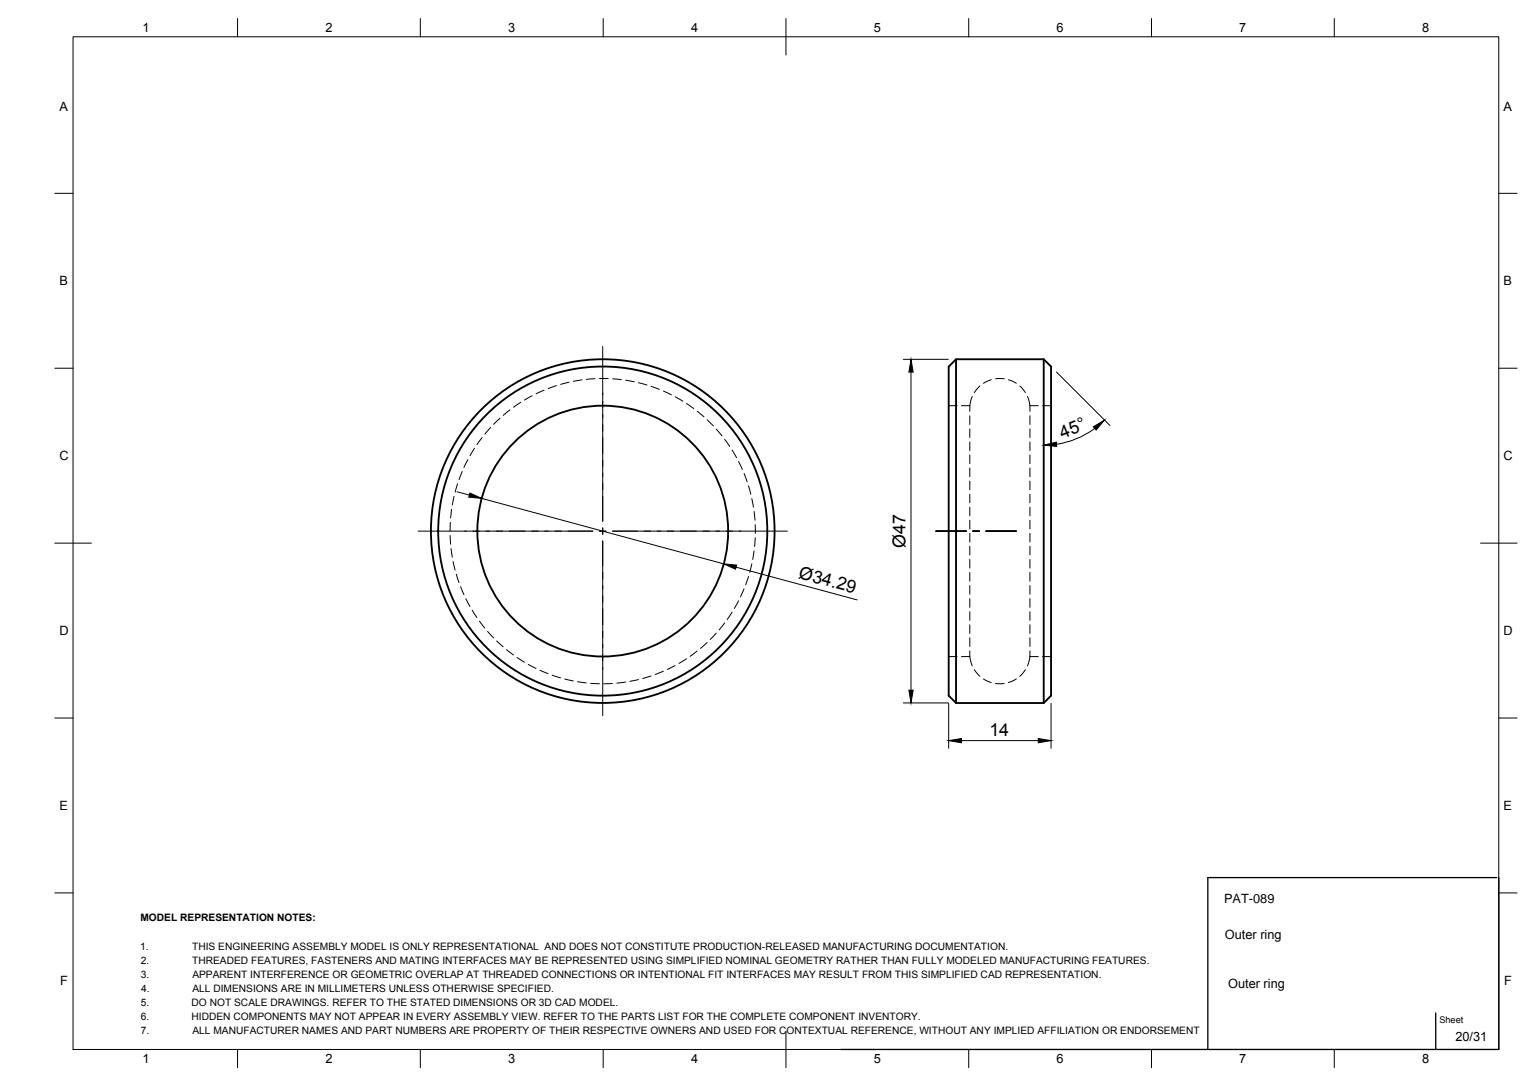
ISO-10303-21;
HEADER;
/* Generated by software containing ST-Developer
 * from STEP Tools, Inc. (www.steptools.com) 
 */

FILE_DESCRIPTION(
/* description */ ('Rotary union on bearing shaft'),
/* implementation_level */ '2;1');

FILE_NAME(
/* name */ 'Outer ring.step',
/* time_stamp */ '2026-10-28T03:24:01-07:00',
/* author */ (''),
/* organization */ (''),
/* preprocessor_version */ 'ST-DEVELOPER v20.2',
/* originating_system */ 'Autodesk Translation Framework v15.17.0.0',
/* authorisation */ '');

FILE_SCHEMA (('AUTOMOTIVE_DESIGN { 1 0 10303 214 3 1 1 }'));
ENDSEC;

DATA;
#10=MECHANICAL_DESIGN_GEOMETRIC_PRESENTATION_REPRESENTATION('',(#325),#9448);
#203=CONICAL_SURFACE('',#5460,2.3,0.785398163397449);
#204=CONICAL_SURFACE('',#5464,2.3,0.785398163397449);
#224=TOROIDAL_SURFACE('',#5449,1.675,0.412776);
#271=SHAPE_REPRESENTATION_RELATIONSHIP('SRR','None',#9572,#298);
#298=ADVANCED_BREP_SHAPE_REPRESENTATION('',(#360),#9432);
#325=STYLED_ITEM('',(#9778),#360);
#360=MANIFOLD_SOLID_BREP('Body1',#4880);
#446=FACE_BOUND('',#1143,.T.);
#447=FACE_BOUND('',#1148,.T.);
#552=PLANE('',#5457);
#553=PLANE('',#5466);
#775=FACE_OUTER_BOUND('',#1140,.T.);
#776=FACE_OUTER_BOUND('',#1141,.T.);
#777=FACE_OUTER_BOUND('',#1142,.T.);
#778=FACE_OUTER_BOUND('',#1144,.T.);
#779=FACE_OUTER_BOUND('',#1145,.T.);
#780=FACE_OUTER_BOUND('',#1146,.T.);
#781=FACE_OUTER_BOUND('',#1147,.T.);
#782=FACE_OUTER_BOUND('',#1149,.T.);
#1140=EDGE_LOOP('',(#3755,#3756,#3757,#3758,#3759,#3760));
#1141=EDGE_LOOP('',(#3761,#3762,#3763,#3764,#3765));
#1142=EDGE_LOOP('',(#3766));
#1143=EDGE_LOOP('',(#3767));
#1144=EDGE_LOOP('',(#3768,#3769,#3770,#3771));
#1145=EDGE_LOOP('',(#3772,#3773,#3774,#3775));
#1146=EDGE_LOOP('',(#3776,#3777,#3778,#3779));
#1147=EDGE_LOOP('',(#3780));
#1148=EDGE_LOOP('',(#3781));
#1149=EDGE_LOOP('',(#3782,#3783,#3784,#3785,#3786));
#1487=LINE('',#8078,#1807);
#1488=LINE('',#8087,#1808);
#1489=LINE('',#8091,#1809);
#1490=LINE('',#8095,#1810);
#1491=LINE('',#8098,#1811);
#1807=VECTOR('',#6460,1.71469);
#1808=VECTOR('',#6471,2.3);
#1809=VECTOR('',#6476,2.35);
#1810=VECTOR('',#6481,2.3);
#1811=VECTOR('',#6486,1.71469);
#2111=CIRCLE('',#5450,1.71469);
#2112=CIRCLE('',#5451,1.71469);
#2113=CIRCLE('',#5452,0.412776);
#2114=CIRCLE('',#5453,1.71469);
#2115=CIRCLE('',#5454,1.71469);
#2116=CIRCLE('',#5456,1.71469);
#2117=CIRCLE('',#5458,2.25);
#2118=CIRCLE('',#5459,1.71469);
#2119=CIRCLE('',#5461,2.35);
#2120=CIRCLE('',#5463,2.35);
#2121=CIRCLE('',#5465,2.25);
#2414=VERTEX_POINT('',#8066);
#2415=VERTEX_POINT('',#8067);
#2416=VERTEX_POINT('',#8070);
#2417=VERTEX_POINT('',#8072);
#2418=VERTEX_POINT('',#8076);
#2419=VERTEX_POINT('',#8080);
#2420=VERTEX_POINT('',#8082);
#2421=VERTEX_POINT('',#8085);
#2422=VERTEX_POINT('',#8089);
#2423=VERTEX_POINT('',#8093);
#2905=EDGE_CURVE('',#2414,#2415,#2111,.T.);
#2906=EDGE_CURVE('',#2415,#2414,#2112,.T.);
#2907=EDGE_CURVE('',#2415,#2416,#2113,.T.);
#2908=EDGE_CURVE('',#2417,#2416,#2114,.T.);
#2909=EDGE_CURVE('',#2416,#2417,#2115,.T.);
#2910=EDGE_CURVE('',#2418,#2418,#2116,.T.);
#2911=EDGE_CURVE('',#2418,#2417,#1487,.T.);
#2912=EDGE_CURVE('',#2419,#2419,#2117,.T.);
#2913=EDGE_CURVE('',#2420,#2420,#2118,.T.);
#2914=EDGE_CURVE('',#2421,#2421,#2119,.T.);
#2915=EDGE_CURVE('',#2421,#2419,#1488,.T.);
#2916=EDGE_CURVE('',#2422,#2422,#2120,.T.);
#2917=EDGE_CURVE('',#2422,#2421,#1489,.T.);
#2918=EDGE_CURVE('',#2423,#2423,#2121,.T.);
#2919=EDGE_CURVE('',#2423,#2422,#1490,.T.);
#2920=EDGE_CURVE('',#2414,#2420,#1491,.T.);
#3755=ORIENTED_EDGE('',*,*,#2905,.F.);
#3756=ORIENTED_EDGE('',*,*,#2906,.F.);
#3757=ORIENTED_EDGE('',*,*,#2907,.T.);
#3758=ORIENTED_EDGE('',*,*,#2908,.F.);
#3759=ORIENTED_EDGE('',*,*,#2909,.F.);
#3760=ORIENTED_EDGE('',*,*,#2907,.F.);
#3761=ORIENTED_EDGE('',*,*,#2910,.T.);
#3762=ORIENTED_EDGE('',*,*,#2911,.T.);
#3763=ORIENTED_EDGE('',*,*,#2908,.T.);
#3764=ORIENTED_EDGE('',*,*,#2909,.T.);
#3765=ORIENTED_EDGE('',*,*,#2911,.F.);
#3766=ORIENTED_EDGE('',*,*,#2912,.F.);
#3767=ORIENTED_EDGE('',*,*,#2913,.T.);
#3768=ORIENTED_EDGE('',*,*,#2914,.F.);
#3769=ORIENTED_EDGE('',*,*,#2915,.T.);
#3770=ORIENTED_EDGE('',*,*,#2912,.T.);
#3771=ORIENTED_EDGE('',*,*,#2915,.F.);
#3772=ORIENTED_EDGE('',*,*,#2916,.F.);
#3773=ORIENTED_EDGE('',*,*,#2917,.T.);
#3774=ORIENTED_EDGE('',*,*,#2914,.T.);
#3775=ORIENTED_EDGE('',*,*,#2917,.F.);
#3776=ORIENTED_EDGE('',*,*,#2918,.F.);
#3777=ORIENTED_EDGE('',*,*,#2919,.T.);
#3778=ORIENTED_EDGE('',*,*,#2916,.T.);
#3779=ORIENTED_EDGE('',*,*,#2919,.F.);
#3780=ORIENTED_EDGE('',*,*,#2918,.T.);
#3781=ORIENTED_EDGE('',*,*,#2910,.F.);
#3782=ORIENTED_EDGE('',*,*,#2905,.T.);
#3783=ORIENTED_EDGE('',*,*,#2906,.T.);
#3784=ORIENTED_EDGE('',*,*,#2920,.T.);
#3785=ORIENTED_EDGE('',*,*,#2913,.F.);
#3786=ORIENTED_EDGE('',*,*,#2920,.F.);
#4528=CYLINDRICAL_SURFACE('',#5455,1.71469);
#4529=CYLINDRICAL_SURFACE('',#5462,2.35);
#4530=CYLINDRICAL_SURFACE('',#5467,1.71469);
#4688=ADVANCED_FACE('',(#775),#224,.F.);
#4689=ADVANCED_FACE('',(#776),#4528,.F.);
#4690=ADVANCED_FACE('',(#777,#446),#552,.T.);
#4691=ADVANCED_FACE('',(#778),#203,.T.);
#4692=ADVANCED_FACE('',(#779),#4529,.T.);
#4693=ADVANCED_FACE('',(#780),#204,.T.);
#4694=ADVANCED_FACE('',(#781,#447),#553,.T.);
#4695=ADVANCED_FACE('',(#782),#4530,.F.);
#4880=CLOSED_SHELL('',(#4688,#4689,#4690,#4691,#4692,#4693,#4694,#4695));
#5448=AXIS2_PLACEMENT_3D('',#8064,#6442,#6443);
#5449=AXIS2_PLACEMENT_3D('',#8065,#6444,#6445);
#5450=AXIS2_PLACEMENT_3D('',#8068,#6446,#6447);
#5451=AXIS2_PLACEMENT_3D('',#8069,#6448,#6449);
#5452=AXIS2_PLACEMENT_3D('',#8071,#6450,#6451);
#5453=AXIS2_PLACEMENT_3D('',#8073,#6452,#6453);
#5454=AXIS2_PLACEMENT_3D('',#8074,#6454,#6455);
#5455=AXIS2_PLACEMENT_3D('',#8075,#6456,#6457);
#5456=AXIS2_PLACEMENT_3D('',#8077,#6458,#6459);
#5457=AXIS2_PLACEMENT_3D('',#8079,#6461,#6462);
#5458=AXIS2_PLACEMENT_3D('',#8081,#6463,#6464);
#5459=AXIS2_PLACEMENT_3D('',#8083,#6465,#6466);
#5460=AXIS2_PLACEMENT_3D('',#8084,#6467,#6468);
#5461=AXIS2_PLACEMENT_3D('',#8086,#6469,#6470);
#5462=AXIS2_PLACEMENT_3D('',#8088,#6472,#6473);
#5463=AXIS2_PLACEMENT_3D('',#8090,#6474,#6475);
#5464=AXIS2_PLACEMENT_3D('',#8092,#6477,#6478);
#5465=AXIS2_PLACEMENT_3D('',#8094,#6479,#6480);
#5466=AXIS2_PLACEMENT_3D('',#8096,#6482,#6483);
#5467=AXIS2_PLACEMENT_3D('',#8097,#6484,#6485);
#6442=DIRECTION('axis',(0.,0.,1.));
#6443=DIRECTION('refdir',(1.,0.,0.));
#6444=DIRECTION('center_axis',(0.,-1.,0.));
#6445=DIRECTION('ref_axis',(0.,0.,-1.));
#6446=DIRECTION('center_axis',(0.,-1.,0.));
#6447=DIRECTION('ref_axis',(1.,0.,0.));
#6448=DIRECTION('center_axis',(0.,-1.,0.));
#6449=DIRECTION('ref_axis',(1.,0.,0.));
#6450=DIRECTION('center_axis',(1.,0.,1.22464679914735E-16));
#6451=DIRECTION('ref_axis',(-1.22464679914735E-16,0.,1.));
#6452=DIRECTION('center_axis',(0.,1.,0.));
#6453=DIRECTION('ref_axis',(1.,0.,0.));
#6454=DIRECTION('center_axis',(0.,1.,0.));
#6455=DIRECTION('ref_axis',(1.,0.,0.));
#6456=DIRECTION('center_axis',(0.,-1.,0.));
#6457=DIRECTION('ref_axis',(1.,0.,0.));
#6458=DIRECTION('center_axis',(0.,-1.,0.));
#6459=DIRECTION('ref_axis',(1.,0.,0.));
#6460=DIRECTION('',(0.,1.,0.));
#6461=DIRECTION('center_axis',(0.,1.,0.));
#6462=DIRECTION('ref_axis',(0.,0.,1.));
#6463=DIRECTION('center_axis',(0.,-1.,0.));
#6464=DIRECTION('ref_axis',(1.,0.,0.));
#6465=DIRECTION('center_axis',(0.,-1.,0.));
#6466=DIRECTION('ref_axis',(1.,0.,0.));
#6467=DIRECTION('center_axis',(0.,-1.,0.));
#6468=DIRECTION('ref_axis',(1.,0.,0.));
#6469=DIRECTION('center_axis',(0.,-1.,0.));
#6470=DIRECTION('ref_axis',(1.,0.,0.));
#6471=DIRECTION('',(0.707106781186548,0.707106781186547,8.65956056235494E-17));
#6472=DIRECTION('center_axis',(0.,-1.,0.));
#6473=DIRECTION('ref_axis',(1.,0.,0.));
#6474=DIRECTION('center_axis',(0.,-1.,0.));
#6475=DIRECTION('ref_axis',(1.,0.,0.));
#6476=DIRECTION('',(0.,1.,0.));
#6477=DIRECTION('center_axis',(0.,1.,0.));
#6478=DIRECTION('ref_axis',(1.,0.,0.));
#6479=DIRECTION('center_axis',(0.,-1.,0.));
#6480=DIRECTION('ref_axis',(1.,0.,0.));
#6481=DIRECTION('',(-0.707106781186548,0.707106781186547,-8.65956056235494E-17));
#6482=DIRECTION('center_axis',(0.,-1.,0.));
#6483=DIRECTION('ref_axis',(0.,0.,-1.));
#6484=DIRECTION('center_axis',(0.,-1.,0.));
#6485=DIRECTION('ref_axis',(1.,0.,0.));
#6486=DIRECTION('',(0.,1.,0.));
#8064=CARTESIAN_POINT('',(0.,0.,0.));
#8065=CARTESIAN_POINT('Origin',(0.,0.,0.));
#8066=CARTESIAN_POINT('',(-1.71469,0.410863395882378,-2.09988962002998E-16));
#8067=CARTESIAN_POINT('',(-2.09988962002998E-16,0.410863395882378,1.71469));
#8068=CARTESIAN_POINT('Origin',(0.,0.410863395882378,0.));
#8069=CARTESIAN_POINT('Origin',(0.,0.410863395882378,0.));
#8070=CARTESIAN_POINT('',(-2.09988962002998E-16,-0.410863395882378,1.71469));
#8071=CARTESIAN_POINT('Origin',(-2.05128338857182E-16,0.,1.675));
#8072=CARTESIAN_POINT('',(-1.71469,-0.410863395882378,2.09988962002998E-16));
#8073=CARTESIAN_POINT('Origin',(0.,-0.410863395882378,0.));
#8074=CARTESIAN_POINT('Origin',(0.,-0.410863395882378,0.));
#8075=CARTESIAN_POINT('Origin',(0.,0.,0.));
#8076=CARTESIAN_POINT('',(-1.71469,-0.7,-2.09988962002998E-16));
#8077=CARTESIAN_POINT('Origin',(0.,-0.7,0.));
#8078=CARTESIAN_POINT('',(-1.71469,0.,-2.09988962002998E-16));
#8079=CARTESIAN_POINT('Origin',(2.25,0.7,0.));
#8080=CARTESIAN_POINT('',(-2.25,0.7,-2.75545529808154E-16));
#8081=CARTESIAN_POINT('Origin',(0.,0.7,0.));
#8082=CARTESIAN_POINT('',(-1.71469,0.7,-2.09988962002998E-16));
#8083=CARTESIAN_POINT('Origin',(0.,0.7,0.));
#8084=CARTESIAN_POINT('Origin',(0.,0.65,0.));
#8085=CARTESIAN_POINT('',(-2.35,0.6,-2.87791997799628E-16));
#8086=CARTESIAN_POINT('Origin',(0.,0.6,0.));
#8087=CARTESIAN_POINT('',(-2.3,0.65,-2.81668763803891E-16));
#8088=CARTESIAN_POINT('Origin',(0.,0.,0.));
#8089=CARTESIAN_POINT('',(-2.35,-0.6,-2.87791997799628E-16));
#8090=CARTESIAN_POINT('Origin',(0.,-0.6,0.));
#8091=CARTESIAN_POINT('',(-2.35,0.,-2.87791997799628E-16));
#8092=CARTESIAN_POINT('Origin',(0.,-0.65,0.));
#8093=CARTESIAN_POINT('',(-2.25,-0.7,-2.75545529808154E-16));
#8094=CARTESIAN_POINT('Origin',(0.,-0.7,0.));
#8095=CARTESIAN_POINT('',(-2.3,-0.65,-2.81668763803891E-16));
#8096=CARTESIAN_POINT('Origin',(1.71469,-0.7,0.));
#8097=CARTESIAN_POINT('Origin',(0.,0.,0.));
#8098=CARTESIAN_POINT('',(-1.71469,0.,-2.09988962002998E-16));
#9400=UNCERTAINTY_MEASURE_WITH_UNIT(LENGTH_MEASURE(0.001),#9449,
'DISTANCE_ACCURACY_VALUE',
'Maximum model space distance between geometric entities at asserted c
onnectivities');
#9416=UNCERTAINTY_MEASURE_WITH_UNIT(LENGTH_MEASURE(0.001),#9449,
'DISTANCE_ACCURACY_VALUE',
'Maximum model space distance between geometric entities at asserted c
onnectivities');
#9432=(
GEOMETRIC_REPRESENTATION_CONTEXT(3)
GLOBAL_UNCERTAINTY_ASSIGNED_CONTEXT((#9400))
GLOBAL_UNIT_ASSIGNED_CONTEXT((#9449,#9451,#9452))
REPRESENTATION_CONTEXT('','3D')
);
#9448=(
GEOMETRIC_REPRESENTATION_CONTEXT(3)
GLOBAL_UNCERTAINTY_ASSIGNED_CONTEXT((#9416))
GLOBAL_UNIT_ASSIGNED_CONTEXT((#9449,#9451,#9452))
REPRESENTATION_CONTEXT('','3D')
);
#9449=(
LENGTH_UNIT()
NAMED_UNIT(*)
SI_UNIT(.CENTI.,.METRE.)
);
#9451=(
NAMED_UNIT(*)
PLANE_ANGLE_UNIT()
SI_UNIT($,.RADIAN.)
);
#9452=(
NAMED_UNIT(*)
SI_UNIT($,.STERADIAN.)
SOLID_ANGLE_UNIT()
);
#9468=SHAPE_DEFINITION_REPRESENTATION(#9499,#9572);
#9499=PRODUCT_DEFINITION_SHAPE('',$,#9604);
#9572=SHAPE_REPRESENTATION('',(#5448),#9432);
#9588=PRODUCT_DEFINITION_CONTEXT('part definition',#9683,'design');
#9604=PRODUCT_DEFINITION('Outer ring','Outer ring',#9635,#9588);
#9635=PRODUCT_DEFINITION_FORMATION('',$,#9700);
#9683=APPLICATION_CONTEXT(
'Core Data for Automotive Mechanical Design Process');
#9684=PRODUCT_CONTEXT('part definition',#9683,'mechanical');
#9700=PRODUCT('Outer ring','Outer ring','Outer ring',(#9684));
#9772=COLOUR_RGB('Grey',0.48,0.52,0.57);
#9773=FILL_AREA_STYLE_COLOUR('',#9772);
#9774=FILL_AREA_STYLE('',(#9773));
#9775=SURFACE_STYLE_FILL_AREA(#9774);
#9776=SURFACE_SIDE_STYLE('',(#9775));
#9777=SURFACE_STYLE_USAGE(.BOTH.,#9776);
#9778=PRESENTATION_STYLE_ASSIGNMENT((#9777));
ENDSEC;
END-ISO-10303-21;
